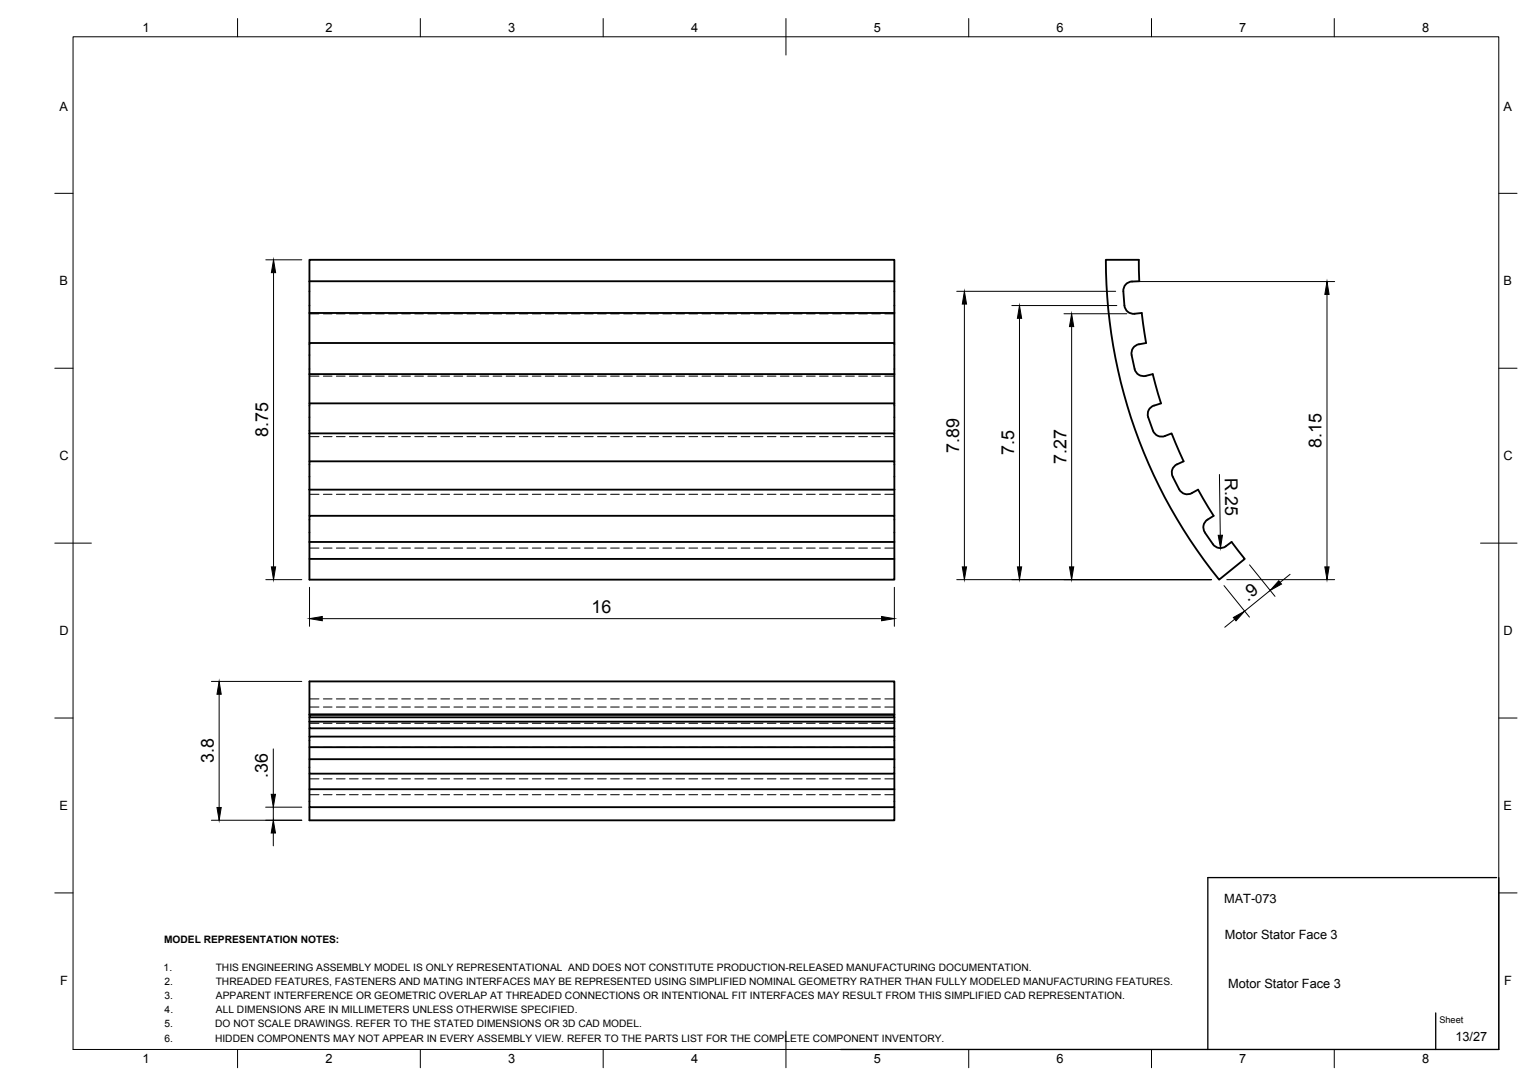
ISO-10303-21;
HEADER;
/* Generated by software containing ST-Developer
 * from STEP Tools, Inc. (www.steptools.com) 
 */

FILE_DESCRIPTION(
/* description */ ('CAx-IF Rec.Pracs.---Representation and Presentation of Product Manufa
cturing Information (PMI)---4.0---2014-10-13'),
/* implementation_level */ '2;1');

FILE_NAME(
/* name */ 'Motor Stator Face 3.step',
/* time_stamp */ '2026-10-24T18:52:33-07:00',
/* author */ (''),
/* organization */ (''),
/* preprocessor_version */ 'ST-DEVELOPER v20.2',
/* originating_system */ 'Autodesk Translation Framework v15.17.0.0',
/* authorisation */ '');

FILE_SCHEMA (('AP242_MANAGED_MODEL_BASED_3D_ENGINEERING_MIM_LF { 1 0 10303 442 2 1 4 }'));
ENDSEC;

DATA;
#10=MECHANICAL_DESIGN_GEOMETRIC_PRESENTATION_REPRESENTATION('',(#426),#34876);
#360=SHAPE_REPRESENTATION_RELATIONSHIP('SRR','None',#34997,#393);
#393=ADVANCED_BREP_SHAPE_REPRESENTATION('',(#459),#34855);
#426=STYLED_ITEM('',(#35163),#459);
#459=MANIFOLD_SOLID_BREP('Motor Stator Face 3',#19566);
#847=PLANE('',#21099);
#848=PLANE('',#21109);
#849=PLANE('',#21119);
#850=PLANE('',#21129);
#851=PLANE('',#21139);
#852=PLANE('',#21140);
#853=PLANE('',#21141);
#854=PLANE('',#21142);
#855=PLANE('',#21143);
#856=PLANE('',#21150);
#857=PLANE('',#21160);
#858=PLANE('',#21163);
#859=PLANE('',#21166);
#860=PLANE('',#21169);
#1841=LINE('',#31602,#3440);
#1842=LINE('',#31605,#3441);
#1843=LINE('',#31610,#3442);
#1844=LINE('',#31616,#3443);
#1845=LINE('',#31620,#3444);
#1846=LINE('',#31622,#3445);
#1847=LINE('',#31623,#3446);
#1848=LINE('',#31629,#3447);
#1849=LINE('',#31632,#3448);
#1850=LINE('',#31637,#3449);
#1851=LINE('',#31643,#3450);
#1852=LINE('',#31647,#3451);
#1853=LINE('',#31649,#3452);
#1854=LINE('',#31650,#3453);
#1855=LINE('',#31656,#3454);
#1856=LINE('',#31659,#3455);
#1857=LINE('',#31664,#3456);
#1858=LINE('',#31670,#3457);
#1859=LINE('',#31674,#3458);
#1860=LINE('',#31676,#3459);
#1861=LINE('',#31677,#3460);
#1862=LINE('',#31683,#3461);
#1863=LINE('',#31686,#3462);
#1864=LINE('',#31691,#3463);
#1865=LINE('',#31697,#3464);
#1866=LINE('',#31701,#3465);
#1867=LINE('',#31703,#3466);
#1868=LINE('',#31704,#3467);
#1869=LINE('',#31710,#3468);
#1870=LINE('',#31713,#3469);
#1871=LINE('',#31718,#3470);
#1872=LINE('',#31724,#3471);
#1873=LINE('',#31728,#3472);
#1874=LINE('',#31730,#3473);
#1875=LINE('',#31731,#3474);
#1876=LINE('',#31734,#3475);
#1877=LINE('',#31736,#3476);
#1878=LINE('',#31737,#3477);
#1879=LINE('',#31740,#3478);
#1880=LINE('',#31742,#3479);
#1881=LINE('',#31743,#3480);
#1882=LINE('',#31746,#3481);
#1883=LINE('',#31748,#3482);
#1884=LINE('',#31749,#3483);
#1885=LINE('',#31752,#3484);
#1886=LINE('',#31754,#3485);
#1887=LINE('',#31755,#3486);
#1888=LINE('',#31760,#3487);
#1889=LINE('',#31767,#3488);
#1890=LINE('',#31771,#3489);
#1891=LINE('',#31776,#3490);
#1892=LINE('',#31781,#3491);
#1893=LINE('',#31784,#3492);
#1894=LINE('',#31787,#3493);
#1895=LINE('',#31792,#3494);
#1896=LINE('',#31793,#3495);
#1897=LINE('',#31797,#3496);
#1898=LINE('',#31799,#3497);
#3440=VECTOR('',#25298,1.);
#3441=VECTOR('',#25301,1.);
#3442=VECTOR('',#25306,1.);
#3443=VECTOR('',#25313,1.);
#3444=VECTOR('',#25318,1.);
#3445=VECTOR('',#25319,1.);
#3446=VECTOR('',#25320,1.);
#3447=VECTOR('',#25325,1.);
#3448=VECTOR('',#25328,1.);
#3449=VECTOR('',#25333,1.);
#3450=VECTOR('',#25340,1.);
#3451=VECTOR('',#25345,1.);
#3452=VECTOR('',#25346,1.);
#3453=VECTOR('',#25347,1.);
#3454=VECTOR('',#25352,1.);
#3455=VECTOR('',#25355,1.);
#3456=VECTOR('',#25360,1.);
#3457=VECTOR('',#25367,1.);
#3458=VECTOR('',#25372,1.);
#3459=VECTOR('',#25373,1.);
#3460=VECTOR('',#25374,1.);
#3461=VECTOR('',#25379,1.);
#3462=VECTOR('',#25382,1.);
#3463=VECTOR('',#25387,1.);
#3464=VECTOR('',#25394,1.);
#3465=VECTOR('',#25399,1.);
#3466=VECTOR('',#25400,1.);
#3467=VECTOR('',#25401,1.);
#3468=VECTOR('',#25406,1.);
#3469=VECTOR('',#25409,1.);
#3470=VECTOR('',#25414,1.);
#3471=VECTOR('',#25421,1.);
#3472=VECTOR('',#25426,1.);
#3473=VECTOR('',#25427,1.);
#3474=VECTOR('',#25428,1.);
#3475=VECTOR('',#25431,1.);
#3476=VECTOR('',#25432,1.);
#3477=VECTOR('',#25433,1.);
#3478=VECTOR('',#25436,1.);
#3479=VECTOR('',#25437,1.);
#3480=VECTOR('',#25438,1.);
#3481=VECTOR('',#25441,1.);
#3482=VECTOR('',#25442,1.);
#3483=VECTOR('',#25443,1.);
#3484=VECTOR('',#25446,1.);
#3485=VECTOR('',#25447,1.);
#3486=VECTOR('',#25448,1.);
#3487=VECTOR('',#25453,1.);
#3488=VECTOR('',#25464,1.);
#3489=VECTOR('',#25467,1.);
#3490=VECTOR('',#25474,1.);
#3491=VECTOR('',#25481,1.);
#3492=VECTOR('',#25484,1.);
#3493=VECTOR('',#25489,1.);
#3494=VECTOR('',#25496,1.);
#3495=VECTOR('',#25497,1.);
#3496=VECTOR('',#25502,1.);
#3497=VECTOR('',#25505,1.);
#4525=CYLINDRICAL_SURFACE('',#21090,0.00025);
#4526=CYLINDRICAL_SURFACE('',#21093,0.01345);
#4527=CYLINDRICAL_SURFACE('',#21096,0.00025);
#4528=CYLINDRICAL_SURFACE('',#21100,0.00025);
#4529=CYLINDRICAL_SURFACE('',#21103,0.01345);
#4530=CYLINDRICAL_SURFACE('',#21106,0.00025);
#4531=CYLINDRICAL_SURFACE('',#21110,0.00025);
#4532=CYLINDRICAL_SURFACE('',#21113,0.01345);
#4533=CYLINDRICAL_SURFACE('',#21116,0.00025);
#4534=CYLINDRICAL_SURFACE('',#21120,0.00025);
#4535=CYLINDRICAL_SURFACE('',#21123,0.01345);
#4536=CYLINDRICAL_SURFACE('',#21126,0.00025);
#4537=CYLINDRICAL_SURFACE('',#21130,0.00025);
#4538=CYLINDRICAL_SURFACE('',#21133,0.01345);
#4539=CYLINDRICAL_SURFACE('',#21136,0.00025);
#4540=CYLINDRICAL_SURFACE('',#21144,0.013);
#4541=CYLINDRICAL_SURFACE('',#21147,0.013);
#4542=CYLINDRICAL_SURFACE('',#21156,0.013);
#4543=CYLINDRICAL_SURFACE('',#21158,0.013);
#4544=CYLINDRICAL_SURFACE('',#21161,0.013);
#4545=CYLINDRICAL_SURFACE('',#21164,0.0139);
#4546=CYLINDRICAL_SURFACE('',#21167,0.013);
#5309=FACE_OUTER_BOUND('',#6408,.T.);
#5310=FACE_OUTER_BOUND('',#6409,.T.);
#5311=FACE_OUTER_BOUND('',#6410,.T.);
#5312=FACE_OUTER_BOUND('',#6411,.T.);
#5313=FACE_OUTER_BOUND('',#6412,.T.);
#5314=FACE_OUTER_BOUND('',#6413,.T.);
#5315=FACE_OUTER_BOUND('',#6414,.T.);
#5316=FACE_OUTER_BOUND('',#6415,.T.);
#5317=FACE_OUTER_BOUND('',#6416,.T.);
#5318=FACE_OUTER_BOUND('',#6417,.T.);
#5319=FACE_OUTER_BOUND('',#6418,.T.);
#5320=FACE_OUTER_BOUND('',#6419,.T.);
#5321=FACE_OUTER_BOUND('',#6420,.T.);
#5322=FACE_OUTER_BOUND('',#6421,.T.);
#5323=FACE_OUTER_BOUND('',#6422,.T.);
#5324=FACE_OUTER_BOUND('',#6423,.T.);
#5325=FACE_OUTER_BOUND('',#6424,.T.);
#5326=FACE_OUTER_BOUND('',#6425,.T.);
#5327=FACE_OUTER_BOUND('',#6426,.T.);
#5328=FACE_OUTER_BOUND('',#6427,.T.);
#5329=FACE_OUTER_BOUND('',#6428,.T.);
#5330=FACE_OUTER_BOUND('',#6429,.T.);
#5331=FACE_OUTER_BOUND('',#6430,.T.);
#5332=FACE_OUTER_BOUND('',#6431,.T.);
#5333=FACE_OUTER_BOUND('',#6432,.T.);
#5334=FACE_OUTER_BOUND('',#6433,.T.);
#5335=FACE_OUTER_BOUND('',#6434,.T.);
#5336=FACE_OUTER_BOUND('',#6435,.T.);
#5337=FACE_OUTER_BOUND('',#6436,.T.);
#5338=FACE_OUTER_BOUND('',#6437,.T.);
#5339=FACE_OUTER_BOUND('',#6438,.T.);
#5340=FACE_OUTER_BOUND('',#6439,.T.);
#5341=FACE_OUTER_BOUND('',#6440,.T.);
#5342=FACE_OUTER_BOUND('',#6441,.T.);
#5343=FACE_OUTER_BOUND('',#6442,.T.);
#5344=FACE_OUTER_BOUND('',#6443,.T.);
#6408=EDGE_LOOP('',(#15580,#15581,#15582,#15583));
#6409=EDGE_LOOP('',(#15584,#15585,#15586,#15587));
#6410=EDGE_LOOP('',(#15588,#15589,#15590,#15591));
#6411=EDGE_LOOP('',(#15592,#15593,#15594,#15595));
#6412=EDGE_LOOP('',(#15596,#15597,#15598,#15599));
#6413=EDGE_LOOP('',(#15600,#15601,#15602,#15603));
#6414=EDGE_LOOP('',(#15604,#15605,#15606,#15607));
#6415=EDGE_LOOP('',(#15608,#15609,#15610,#15611));
#6416=EDGE_LOOP('',(#15612,#15613,#15614,#15615));
#6417=EDGE_LOOP('',(#15616,#15617,#15618,#15619));
#6418=EDGE_LOOP('',(#15620,#15621,#15622,#15623));
#6419=EDGE_LOOP('',(#15624,#15625,#15626,#15627));
#6420=EDGE_LOOP('',(#15628,#15629,#15630,#15631));
#6421=EDGE_LOOP('',(#15632,#15633,#15634,#15635));
#6422=EDGE_LOOP('',(#15636,#15637,#15638,#15639));
#6423=EDGE_LOOP('',(#15640,#15641,#15642,#15643));
#6424=EDGE_LOOP('',(#15644,#15645,#15646,#15647));
#6425=EDGE_LOOP('',(#15648,#15649,#15650,#15651));
#6426=EDGE_LOOP('',(#15652,#15653,#15654,#15655));
#6427=EDGE_LOOP('',(#15656,#15657,#15658,#15659));
#6428=EDGE_LOOP('',(#15660,#15661,#15662,#15663));
#6429=EDGE_LOOP('',(#15664,#15665,#15666,#15667));
#6430=EDGE_LOOP('',(#15668,#15669,#15670,#15671));
#6431=EDGE_LOOP('',(#15672,#15673,#15674,#15675));
#6432=EDGE_LOOP('',(#15676,#15677,#15678,#15679));
#6433=EDGE_LOOP('',(#15680,#15681,#15682,#15683));
#6434=EDGE_LOOP('',(#15684,#15685,#15686,#15687,#15688,#15689,#15690,#15691,
#15692,#15693,#15694,#15695,#15696,#15697,#15698,#15699,#15700,#15701,#15702,
#15703,#15704,#15705,#15706,#15707,#15708,#15709,#15710,#15711,#15712,#15713,
#15714,#15715,#15716,#15717));
#6435=EDGE_LOOP('',(#15718,#15719,#15720,#15721));
#6436=EDGE_LOOP('',(#15722,#15723,#15724,#15725));
#6437=EDGE_LOOP('',(#15726,#15727,#15728,#15729));
#6438=EDGE_LOOP('',(#15730,#15731,#15732,#15733));
#6439=EDGE_LOOP('',(#15734,#15735,#15736,#15737));
#6440=EDGE_LOOP('',(#15738,#15739,#15740,#15741));
#6441=EDGE_LOOP('',(#15742,#15743,#15744,#15745));
#6442=EDGE_LOOP('',(#15746,#15747,#15748,#15749));
#6443=EDGE_LOOP('',(#15750,#15751,#15752,#15753,#15754,#15755,#15756,#15757,
#15758,#15759,#15760,#15761,#15762,#15763,#15764,#15765,#15766,#15767,#15768,
#15769,#15770,#15771,#15772,#15773,#15774,#15775,#15776,#15777,#15778,#15779,
#15780,#15781,#15782,#15783));
#7490=CIRCLE('',#21091,0.000250000000013569);
#7491=CIRCLE('',#21092,0.000250000000013569);
#7492=CIRCLE('',#21094,0.0134500000000125);
#7493=CIRCLE('',#21095,0.0134500000000125);
#7494=CIRCLE('',#21097,0.000250000000013744);
#7495=CIRCLE('',#21098,0.000250000000013744);
#7496=CIRCLE('',#21101,0.000250000000013973);
#7497=CIRCLE('',#21102,0.000250000000013973);
#7498=CIRCLE('',#21104,0.0134500000000115);
#7499=CIRCLE('',#21105,0.0134500000000115);
#7500=CIRCLE('',#21107,0.000250000000014062);
#7501=CIRCLE('',#21108,0.000250000000014062);
#7502=CIRCLE('',#21111,0.000250000000014138);
#7503=CIRCLE('',#21112,0.000250000000014138);
#7504=CIRCLE('',#21114,0.0134500000000103);
#7505=CIRCLE('',#21115,0.0134500000000103);
#7506=CIRCLE('',#21117,0.000250000000014138);
#7507=CIRCLE('',#21118,0.000250000000014138);
#7508=CIRCLE('',#21121,0.000250000000014062);
#7509=CIRCLE('',#21122,0.000250000000014062);
#7510=CIRCLE('',#21124,0.0134500000000109);
#7511=CIRCLE('',#21125,0.0134500000000109);
#7512=CIRCLE('',#21127,0.000250000000013973);
#7513=CIRCLE('',#21128,0.000250000000013973);
#7514=CIRCLE('',#21131,0.000250000000013744);
#7515=CIRCLE('',#21132,0.000250000000013744);
#7516=CIRCLE('',#21134,0.013450000000012);
#7517=CIRCLE('',#21135,0.013450000000012);
#7518=CIRCLE('',#21137,0.000250000000013569);
#7519=CIRCLE('',#21138,0.000250000000013569);
#7520=CIRCLE('',#21145,0.0130000000000128);
#7521=CIRCLE('',#21146,0.0130000000000128);
#7522=CIRCLE('',#21148,0.0130000000000128);
#7523=CIRCLE('',#21149,0.0130000000000128);
#7524=CIRCLE('',#21151,0.0139000000000128);
#7525=CIRCLE('',#21152,0.0130000000000128);
#7526=CIRCLE('',#21153,0.0130000000000128);
#7527=CIRCLE('',#21154,0.0130000000000128);
#7528=CIRCLE('',#21155,0.0130000000000128);
#7529=CIRCLE('',#21157,0.0130000000000128);
#7530=CIRCLE('',#21159,0.0130000000000128);
#7531=CIRCLE('',#21162,0.0130000000000128);
#7532=CIRCLE('',#21165,0.0139000000000128);
#7533=CIRCLE('',#21168,0.0130000000000128);
#8990=VERTEX_POINT('',#31598);
#8991=VERTEX_POINT('',#31599);
#8992=VERTEX_POINT('',#31601);
#8993=VERTEX_POINT('',#31603);
#8994=VERTEX_POINT('',#31607);
#8995=VERTEX_POINT('',#31609);
#8996=VERTEX_POINT('',#31613);
#8997=VERTEX_POINT('',#31615);
#8998=VERTEX_POINT('',#31619);
#8999=VERTEX_POINT('',#31621);
#9000=VERTEX_POINT('',#31625);
#9001=VERTEX_POINT('',#31626);
#9002=VERTEX_POINT('',#31628);
#9003=VERTEX_POINT('',#31630);
#9004=VERTEX_POINT('',#31634);
#9005=VERTEX_POINT('',#31636);
#9006=VERTEX_POINT('',#31640);
#9007=VERTEX_POINT('',#31642);
#9008=VERTEX_POINT('',#31646);
#9009=VERTEX_POINT('',#31648);
#9010=VERTEX_POINT('',#31652);
#9011=VERTEX_POINT('',#31653);
#9012=VERTEX_POINT('',#31655);
#9013=VERTEX_POINT('',#31657);
#9014=VERTEX_POINT('',#31661);
#9015=VERTEX_POINT('',#31663);
#9016=VERTEX_POINT('',#31667);
#9017=VERTEX_POINT('',#31669);
#9018=VERTEX_POINT('',#31673);
#9019=VERTEX_POINT('',#31675);
#9020=VERTEX_POINT('',#31679);
#9021=VERTEX_POINT('',#31680);
#9022=VERTEX_POINT('',#31682);
#9023=VERTEX_POINT('',#31684);
#9024=VERTEX_POINT('',#31688);
#9025=VERTEX_POINT('',#31690);
#9026=VERTEX_POINT('',#31694);
#9027=VERTEX_POINT('',#31696);
#9028=VERTEX_POINT('',#31700);
#9029=VERTEX_POINT('',#31702);
#9030=VERTEX_POINT('',#31706);
#9031=VERTEX_POINT('',#31707);
#9032=VERTEX_POINT('',#31709);
#9033=VERTEX_POINT('',#31711);
#9034=VERTEX_POINT('',#31715);
#9035=VERTEX_POINT('',#31717);
#9036=VERTEX_POINT('',#31721);
#9037=VERTEX_POINT('',#31723);
#9038=VERTEX_POINT('',#31727);
#9039=VERTEX_POINT('',#31729);
#9040=VERTEX_POINT('',#31733);
#9041=VERTEX_POINT('',#31735);
#9042=VERTEX_POINT('',#31739);
#9043=VERTEX_POINT('',#31741);
#9044=VERTEX_POINT('',#31745);
#9045=VERTEX_POINT('',#31747);
#9046=VERTEX_POINT('',#31751);
#9047=VERTEX_POINT('',#31753);
#9048=VERTEX_POINT('',#31757);
#9049=VERTEX_POINT('',#31759);
#9050=VERTEX_POINT('',#31766);
#9051=VERTEX_POINT('',#31768);
#9052=VERTEX_POINT('',#31770);
#9053=VERTEX_POINT('',#31774);
#9054=VERTEX_POINT('',#31779);
#9055=VERTEX_POINT('',#31783);
#9056=VERTEX_POINT('',#31791);
#9057=VERTEX_POINT('',#31795);
#11348=EDGE_CURVE('',#8990,#8991,#7490,.T.);
#11349=EDGE_CURVE('',#8991,#8992,#1841,.T.);
#11350=EDGE_CURVE('',#8992,#8993,#7491,.T.);
#11351=EDGE_CURVE('',#8993,#8990,#1842,.T.);
#11352=EDGE_CURVE('',#8994,#8991,#7492,.T.);
#11353=EDGE_CURVE('',#8995,#8994,#1843,.T.);
#11354=EDGE_CURVE('',#8992,#8995,#7493,.T.);
#11355=EDGE_CURVE('',#8994,#8996,#7494,.T.);
#11356=EDGE_CURVE('',#8996,#8997,#1844,.T.);
#11357=EDGE_CURVE('',#8997,#8995,#7495,.T.);
#11358=EDGE_CURVE('',#8998,#8996,#1845,.T.);
#11359=EDGE_CURVE('',#8999,#8998,#1846,.T.);
#11360=EDGE_CURVE('',#8997,#8999,#1847,.T.);
#11361=EDGE_CURVE('',#9000,#9001,#7496,.T.);
#11362=EDGE_CURVE('',#9001,#9002,#1848,.T.);
#11363=EDGE_CURVE('',#9002,#9003,#7497,.T.);
#11364=EDGE_CURVE('',#9003,#9000,#1849,.T.);
#11365=EDGE_CURVE('',#9004,#9001,#7498,.T.);
#11366=EDGE_CURVE('',#9005,#9004,#1850,.T.);
#11367=EDGE_CURVE('',#9002,#9005,#7499,.T.);
#11368=EDGE_CURVE('',#9004,#9006,#7500,.T.);
#11369=EDGE_CURVE('',#9006,#9007,#1851,.T.);
#11370=EDGE_CURVE('',#9007,#9005,#7501,.T.);
#11371=EDGE_CURVE('',#9008,#9006,#1852,.T.);
#11372=EDGE_CURVE('',#9009,#9008,#1853,.T.);
#11373=EDGE_CURVE('',#9007,#9009,#1854,.T.);
#11374=EDGE_CURVE('',#9010,#9011,#7502,.T.);
#11375=EDGE_CURVE('',#9011,#9012,#1855,.T.);
#11376=EDGE_CURVE('',#9012,#9013,#7503,.T.);
#11377=EDGE_CURVE('',#9013,#9010,#1856,.T.);
#11378=EDGE_CURVE('',#9014,#9011,#7504,.T.);
#11379=EDGE_CURVE('',#9015,#9014,#1857,.T.);
#11380=EDGE_CURVE('',#9012,#9015,#7505,.T.);
#11381=EDGE_CURVE('',#9014,#9016,#7506,.T.);
#11382=EDGE_CURVE('',#9016,#9017,#1858,.T.);
#11383=EDGE_CURVE('',#9017,#9015,#7507,.T.);
#11384=EDGE_CURVE('',#9018,#9016,#1859,.T.);
#11385=EDGE_CURVE('',#9019,#9018,#1860,.T.);
#11386=EDGE_CURVE('',#9017,#9019,#1861,.T.);
#11387=EDGE_CURVE('',#9020,#9021,#7508,.T.);
#11388=EDGE_CURVE('',#9021,#9022,#1862,.T.);
#11389=EDGE_CURVE('',#9022,#9023,#7509,.T.);
#11390=EDGE_CURVE('',#9023,#9020,#1863,.T.);
#11391=EDGE_CURVE('',#9024,#9021,#7510,.T.);
#11392=EDGE_CURVE('',#9025,#9024,#1864,.T.);
#11393=EDGE_CURVE('',#9022,#9025,#7511,.T.);
#11394=EDGE_CURVE('',#9024,#9026,#7512,.T.);
#11395=EDGE_CURVE('',#9026,#9027,#1865,.T.);
#11396=EDGE_CURVE('',#9027,#9025,#7513,.T.);
#11397=EDGE_CURVE('',#9028,#9026,#1866,.T.);
#11398=EDGE_CURVE('',#9029,#9028,#1867,.T.);
#11399=EDGE_CURVE('',#9027,#9029,#1868,.T.);
#11400=EDGE_CURVE('',#9030,#9031,#7514,.T.);
#11401=EDGE_CURVE('',#9031,#9032,#1869,.T.);
#11402=EDGE_CURVE('',#9032,#9033,#7515,.T.);
#11403=EDGE_CURVE('',#9033,#9030,#1870,.T.);
#11404=EDGE_CURVE('',#9034,#9031,#7516,.T.);
#11405=EDGE_CURVE('',#9035,#9034,#1871,.T.);
#11406=EDGE_CURVE('',#9032,#9035,#7517,.T.);
#11407=EDGE_CURVE('',#9034,#9036,#7518,.T.);
#11408=EDGE_CURVE('',#9036,#9037,#1872,.T.);
#11409=EDGE_CURVE('',#9037,#9035,#7519,.T.);
#11410=EDGE_CURVE('',#9038,#9036,#1873,.T.);
#11411=EDGE_CURVE('',#9039,#9038,#1874,.T.);
#11412=EDGE_CURVE('',#9037,#9039,#1875,.T.);
#11413=EDGE_CURVE('',#9040,#9033,#1876,.T.);
#11414=EDGE_CURVE('',#9041,#9040,#1877,.T.);
#11415=EDGE_CURVE('',#9030,#9041,#1878,.T.);
#11416=EDGE_CURVE('',#9042,#9023,#1879,.T.);
#11417=EDGE_CURVE('',#9043,#9042,#1880,.T.);
#11418=EDGE_CURVE('',#9020,#9043,#1881,.T.);
#11419=EDGE_CURVE('',#9044,#9003,#1882,.T.);
#11420=EDGE_CURVE('',#9045,#9044,#1883,.T.);
#11421=EDGE_CURVE('',#9000,#9045,#1884,.T.);
#11422=EDGE_CURVE('',#9046,#8993,#1885,.T.);
#11423=EDGE_CURVE('',#9047,#9046,#1886,.T.);
#11424=EDGE_CURVE('',#8990,#9047,#1887,.T.);
#11425=EDGE_CURVE('',#9048,#9038,#7520,.T.);
#11426=EDGE_CURVE('',#9048,#9049,#1888,.T.);
#11427=EDGE_CURVE('',#9039,#9049,#7521,.T.);
#11428=EDGE_CURVE('',#9019,#9042,#7522,.T.);
#11429=EDGE_CURVE('',#9043,#9018,#7523,.T.);
#11430=EDGE_CURVE('',#9049,#9050,#1889,.T.);
#11431=EDGE_CURVE('',#9050,#9051,#7524,.T.);
#11432=EDGE_CURVE('',#9051,#9052,#1890,.T.);
#11433=EDGE_CURVE('',#9052,#9046,#7525,.T.);
#11434=EDGE_CURVE('',#8999,#9044,#7526,.T.);
#11435=EDGE_CURVE('',#9009,#9053,#7527,.T.);
#11436=EDGE_CURVE('',#9053,#9013,#1891,.T.);
#11437=EDGE_CURVE('',#9029,#9040,#7528,.T.);
#11438=EDGE_CURVE('',#9054,#9008,#7529,.T.);
#11439=EDGE_CURVE('',#9054,#9053,#1892,.T.);
#11440=EDGE_CURVE('',#9052,#9055,#1893,.T.);
#11441=EDGE_CURVE('',#9047,#9055,#7530,.T.);
#11442=EDGE_CURVE('',#9010,#9054,#1894,.T.);
#11443=EDGE_CURVE('',#9041,#9028,#7531,.T.);
#11444=EDGE_CURVE('',#9056,#9048,#1895,.T.);
#11445=EDGE_CURVE('',#9050,#9056,#1896,.T.);
#11446=EDGE_CURVE('',#9057,#9056,#7532,.T.);
#11447=EDGE_CURVE('',#9051,#9057,#1897,.T.);
#11448=EDGE_CURVE('',#9055,#9057,#1898,.T.);
#11449=EDGE_CURVE('',#9045,#8998,#7533,.T.);
#15580=ORIENTED_EDGE('',*,*,#11348,.T.);
#15581=ORIENTED_EDGE('',*,*,#11349,.T.);
#15582=ORIENTED_EDGE('',*,*,#11350,.T.);
#15583=ORIENTED_EDGE('',*,*,#11351,.T.);
#15584=ORIENTED_EDGE('',*,*,#11349,.F.);
#15585=ORIENTED_EDGE('',*,*,#11352,.F.);
#15586=ORIENTED_EDGE('',*,*,#11353,.F.);
#15587=ORIENTED_EDGE('',*,*,#11354,.F.);
#15588=ORIENTED_EDGE('',*,*,#11355,.T.);
#15589=ORIENTED_EDGE('',*,*,#11356,.T.);
#15590=ORIENTED_EDGE('',*,*,#11357,.T.);
#15591=ORIENTED_EDGE('',*,*,#11353,.T.);
#15592=ORIENTED_EDGE('',*,*,#11356,.F.);
#15593=ORIENTED_EDGE('',*,*,#11358,.F.);
#15594=ORIENTED_EDGE('',*,*,#11359,.F.);
#15595=ORIENTED_EDGE('',*,*,#11360,.F.);
#15596=ORIENTED_EDGE('',*,*,#11361,.T.);
#15597=ORIENTED_EDGE('',*,*,#11362,.T.);
#15598=ORIENTED_EDGE('',*,*,#11363,.T.);
#15599=ORIENTED_EDGE('',*,*,#11364,.T.);
#15600=ORIENTED_EDGE('',*,*,#11362,.F.);
#15601=ORIENTED_EDGE('',*,*,#11365,.F.);
#15602=ORIENTED_EDGE('',*,*,#11366,.F.);
#15603=ORIENTED_EDGE('',*,*,#11367,.F.);
#15604=ORIENTED_EDGE('',*,*,#11368,.T.);
#15605=ORIENTED_EDGE('',*,*,#11369,.T.);
#15606=ORIENTED_EDGE('',*,*,#11370,.T.);
#15607=ORIENTED_EDGE('',*,*,#11366,.T.);
#15608=ORIENTED_EDGE('',*,*,#11369,.F.);
#15609=ORIENTED_EDGE('',*,*,#11371,.F.);
#15610=ORIENTED_EDGE('',*,*,#11372,.F.);
#15611=ORIENTED_EDGE('',*,*,#11373,.F.);
#15612=ORIENTED_EDGE('',*,*,#11374,.T.);
#15613=ORIENTED_EDGE('',*,*,#11375,.T.);
#15614=ORIENTED_EDGE('',*,*,#11376,.T.);
#15615=ORIENTED_EDGE('',*,*,#11377,.T.);
#15616=ORIENTED_EDGE('',*,*,#11375,.F.);
#15617=ORIENTED_EDGE('',*,*,#11378,.F.);
#15618=ORIENTED_EDGE('',*,*,#11379,.F.);
#15619=ORIENTED_EDGE('',*,*,#11380,.F.);
#15620=ORIENTED_EDGE('',*,*,#11381,.T.);
#15621=ORIENTED_EDGE('',*,*,#11382,.T.);
#15622=ORIENTED_EDGE('',*,*,#11383,.T.);
#15623=ORIENTED_EDGE('',*,*,#11379,.T.);
#15624=ORIENTED_EDGE('',*,*,#11382,.F.);
#15625=ORIENTED_EDGE('',*,*,#11384,.F.);
#15626=ORIENTED_EDGE('',*,*,#11385,.F.);
#15627=ORIENTED_EDGE('',*,*,#11386,.F.);
#15628=ORIENTED_EDGE('',*,*,#11387,.T.);
#15629=ORIENTED_EDGE('',*,*,#11388,.T.);
#15630=ORIENTED_EDGE('',*,*,#11389,.T.);
#15631=ORIENTED_EDGE('',*,*,#11390,.T.);
#15632=ORIENTED_EDGE('',*,*,#11388,.F.);
#15633=ORIENTED_EDGE('',*,*,#11391,.F.);
#15634=ORIENTED_EDGE('',*,*,#11392,.F.);
#15635=ORIENTED_EDGE('',*,*,#11393,.F.);
#15636=ORIENTED_EDGE('',*,*,#11394,.T.);
#15637=ORIENTED_EDGE('',*,*,#11395,.T.);
#15638=ORIENTED_EDGE('',*,*,#11396,.T.);
#15639=ORIENTED_EDGE('',*,*,#11392,.T.);
#15640=ORIENTED_EDGE('',*,*,#11395,.F.);
#15641=ORIENTED_EDGE('',*,*,#11397,.F.);
#15642=ORIENTED_EDGE('',*,*,#11398,.F.);
#15643=ORIENTED_EDGE('',*,*,#11399,.F.);
#15644=ORIENTED_EDGE('',*,*,#11400,.T.);
#15645=ORIENTED_EDGE('',*,*,#11401,.T.);
#15646=ORIENTED_EDGE('',*,*,#11402,.T.);
#15647=ORIENTED_EDGE('',*,*,#11403,.T.);
#15648=ORIENTED_EDGE('',*,*,#11401,.F.);
#15649=ORIENTED_EDGE('',*,*,#11404,.F.);
#15650=ORIENTED_EDGE('',*,*,#11405,.F.);
#15651=ORIENTED_EDGE('',*,*,#11406,.F.);
#15652=ORIENTED_EDGE('',*,*,#11407,.T.);
#15653=ORIENTED_EDGE('',*,*,#11408,.T.);
#15654=ORIENTED_EDGE('',*,*,#11409,.T.);
#15655=ORIENTED_EDGE('',*,*,#11405,.T.);
#15656=ORIENTED_EDGE('',*,*,#11408,.F.);
#15657=ORIENTED_EDGE('',*,*,#11410,.F.);
#15658=ORIENTED_EDGE('',*,*,#11411,.F.);
#15659=ORIENTED_EDGE('',*,*,#11412,.F.);
#15660=ORIENTED_EDGE('',*,*,#11403,.F.);
#15661=ORIENTED_EDGE('',*,*,#11413,.F.);
#15662=ORIENTED_EDGE('',*,*,#11414,.F.);
#15663=ORIENTED_EDGE('',*,*,#11415,.F.);
#15664=ORIENTED_EDGE('',*,*,#11390,.F.);
#15665=ORIENTED_EDGE('',*,*,#11416,.F.);
#15666=ORIENTED_EDGE('',*,*,#11417,.F.);
#15667=ORIENTED_EDGE('',*,*,#11418,.F.);
#15668=ORIENTED_EDGE('',*,*,#11364,.F.);
#15669=ORIENTED_EDGE('',*,*,#11419,.F.);
#15670=ORIENTED_EDGE('',*,*,#11420,.F.);
#15671=ORIENTED_EDGE('',*,*,#11421,.F.);
#15672=ORIENTED_EDGE('',*,*,#11351,.F.);
#15673=ORIENTED_EDGE('',*,*,#11422,.F.);
#15674=ORIENTED_EDGE('',*,*,#11423,.F.);
#15675=ORIENTED_EDGE('',*,*,#11424,.F.);
#15676=ORIENTED_EDGE('',*,*,#11411,.T.);
#15677=ORIENTED_EDGE('',*,*,#11425,.F.);
#15678=ORIENTED_EDGE('',*,*,#11426,.T.);
#15679=ORIENTED_EDGE('',*,*,#11427,.F.);
#15680=ORIENTED_EDGE('',*,*,#11417,.T.);
#15681=ORIENTED_EDGE('',*,*,#11428,.F.);
#15682=ORIENTED_EDGE('',*,*,#11385,.T.);
#15683=ORIENTED_EDGE('',*,*,#11429,.F.);
#15684=ORIENTED_EDGE('',*,*,#11413,.T.);
#15685=ORIENTED_EDGE('',*,*,#11402,.F.);
#15686=ORIENTED_EDGE('',*,*,#11406,.T.);
#15687=ORIENTED_EDGE('',*,*,#11409,.F.);
#15688=ORIENTED_EDGE('',*,*,#11412,.T.);
#15689=ORIENTED_EDGE('',*,*,#11427,.T.);
#15690=ORIENTED_EDGE('',*,*,#11430,.T.);
#15691=ORIENTED_EDGE('',*,*,#11431,.T.);
#15692=ORIENTED_EDGE('',*,*,#11432,.T.);
#15693=ORIENTED_EDGE('',*,*,#11433,.T.);
#15694=ORIENTED_EDGE('',*,*,#11422,.T.);
#15695=ORIENTED_EDGE('',*,*,#11350,.F.);
#15696=ORIENTED_EDGE('',*,*,#11354,.T.);
#15697=ORIENTED_EDGE('',*,*,#11357,.F.);
#15698=ORIENTED_EDGE('',*,*,#11360,.T.);
#15699=ORIENTED_EDGE('',*,*,#11434,.T.);
#15700=ORIENTED_EDGE('',*,*,#11419,.T.);
#15701=ORIENTED_EDGE('',*,*,#11363,.F.);
#15702=ORIENTED_EDGE('',*,*,#11367,.T.);
#15703=ORIENTED_EDGE('',*,*,#11370,.F.);
#15704=ORIENTED_EDGE('',*,*,#11373,.T.);
#15705=ORIENTED_EDGE('',*,*,#11435,.T.);
#15706=ORIENTED_EDGE('',*,*,#11436,.T.);
#15707=ORIENTED_EDGE('',*,*,#11376,.F.);
#15708=ORIENTED_EDGE('',*,*,#11380,.T.);
#15709=ORIENTED_EDGE('',*,*,#11383,.F.);
#15710=ORIENTED_EDGE('',*,*,#11386,.T.);
#15711=ORIENTED_EDGE('',*,*,#11428,.T.);
#15712=ORIENTED_EDGE('',*,*,#11416,.T.);
#15713=ORIENTED_EDGE('',*,*,#11389,.F.);
#15714=ORIENTED_EDGE('',*,*,#11393,.T.);
#15715=ORIENTED_EDGE('',*,*,#11396,.F.);
#15716=ORIENTED_EDGE('',*,*,#11399,.T.);
#15717=ORIENTED_EDGE('',*,*,#11437,.T.);
#15718=ORIENTED_EDGE('',*,*,#11372,.T.);
#15719=ORIENTED_EDGE('',*,*,#11438,.F.);
#15720=ORIENTED_EDGE('',*,*,#11439,.T.);
#15721=ORIENTED_EDGE('',*,*,#11435,.F.);
#15722=ORIENTED_EDGE('',*,*,#11423,.T.);
#15723=ORIENTED_EDGE('',*,*,#11433,.F.);
#15724=ORIENTED_EDGE('',*,*,#11440,.T.);
#15725=ORIENTED_EDGE('',*,*,#11441,.F.);
#15726=ORIENTED_EDGE('',*,*,#11377,.F.);
#15727=ORIENTED_EDGE('',*,*,#11436,.F.);
#15728=ORIENTED_EDGE('',*,*,#11439,.F.);
#15729=ORIENTED_EDGE('',*,*,#11442,.F.);
#15730=ORIENTED_EDGE('',*,*,#11414,.T.);
#15731=ORIENTED_EDGE('',*,*,#11437,.F.);
#15732=ORIENTED_EDGE('',*,*,#11398,.T.);
#15733=ORIENTED_EDGE('',*,*,#11443,.F.);
#15734=ORIENTED_EDGE('',*,*,#11426,.F.);
#15735=ORIENTED_EDGE('',*,*,#11444,.F.);
#15736=ORIENTED_EDGE('',*,*,#11445,.F.);
#15737=ORIENTED_EDGE('',*,*,#11430,.F.);
#15738=ORIENTED_EDGE('',*,*,#11445,.T.);
#15739=ORIENTED_EDGE('',*,*,#11446,.F.);
#15740=ORIENTED_EDGE('',*,*,#11447,.F.);
#15741=ORIENTED_EDGE('',*,*,#11431,.F.);
#15742=ORIENTED_EDGE('',*,*,#11447,.T.);
#15743=ORIENTED_EDGE('',*,*,#11448,.F.);
#15744=ORIENTED_EDGE('',*,*,#11440,.F.);
#15745=ORIENTED_EDGE('',*,*,#11432,.F.);
#15746=ORIENTED_EDGE('',*,*,#11420,.T.);
#15747=ORIENTED_EDGE('',*,*,#11434,.F.);
#15748=ORIENTED_EDGE('',*,*,#11359,.T.);
#15749=ORIENTED_EDGE('',*,*,#11449,.F.);
#15750=ORIENTED_EDGE('',*,*,#11415,.T.);
#15751=ORIENTED_EDGE('',*,*,#11443,.T.);
#15752=ORIENTED_EDGE('',*,*,#11397,.T.);
#15753=ORIENTED_EDGE('',*,*,#11394,.F.);
#15754=ORIENTED_EDGE('',*,*,#11391,.T.);
#15755=ORIENTED_EDGE('',*,*,#11387,.F.);
#15756=ORIENTED_EDGE('',*,*,#11418,.T.);
#15757=ORIENTED_EDGE('',*,*,#11429,.T.);
#15758=ORIENTED_EDGE('',*,*,#11384,.T.);
#15759=ORIENTED_EDGE('',*,*,#11381,.F.);
#15760=ORIENTED_EDGE('',*,*,#11378,.T.);
#15761=ORIENTED_EDGE('',*,*,#11374,.F.);
#15762=ORIENTED_EDGE('',*,*,#11442,.T.);
#15763=ORIENTED_EDGE('',*,*,#11438,.T.);
#15764=ORIENTED_EDGE('',*,*,#11371,.T.);
#15765=ORIENTED_EDGE('',*,*,#11368,.F.);
#15766=ORIENTED_EDGE('',*,*,#11365,.T.);
#15767=ORIENTED_EDGE('',*,*,#11361,.F.);
#15768=ORIENTED_EDGE('',*,*,#11421,.T.);
#15769=ORIENTED_EDGE('',*,*,#11449,.T.);
#15770=ORIENTED_EDGE('',*,*,#11358,.T.);
#15771=ORIENTED_EDGE('',*,*,#11355,.F.);
#15772=ORIENTED_EDGE('',*,*,#11352,.T.);
#15773=ORIENTED_EDGE('',*,*,#11348,.F.);
#15774=ORIENTED_EDGE('',*,*,#11424,.T.);
#15775=ORIENTED_EDGE('',*,*,#11441,.T.);
#15776=ORIENTED_EDGE('',*,*,#11448,.T.);
#15777=ORIENTED_EDGE('',*,*,#11446,.T.);
#15778=ORIENTED_EDGE('',*,*,#11444,.T.);
#15779=ORIENTED_EDGE('',*,*,#11425,.T.);
#15780=ORIENTED_EDGE('',*,*,#11410,.T.);
#15781=ORIENTED_EDGE('',*,*,#11407,.F.);
#15782=ORIENTED_EDGE('',*,*,#11404,.T.);
#15783=ORIENTED_EDGE('',*,*,#11400,.F.);
#19025=ADVANCED_FACE('',(#5309),#4525,.F.);
#19026=ADVANCED_FACE('',(#5310),#4526,.F.);
#19027=ADVANCED_FACE('',(#5311),#4527,.F.);
#19028=ADVANCED_FACE('',(#5312),#847,.F.);
#19029=ADVANCED_FACE('',(#5313),#4528,.F.);
#19030=ADVANCED_FACE('',(#5314),#4529,.F.);
#19031=ADVANCED_FACE('',(#5315),#4530,.F.);
#19032=ADVANCED_FACE('',(#5316),#848,.F.);
#19033=ADVANCED_FACE('',(#5317),#4531,.F.);
#19034=ADVANCED_FACE('',(#5318),#4532,.F.);
#19035=ADVANCED_FACE('',(#5319),#4533,.F.);
#19036=ADVANCED_FACE('',(#5320),#849,.F.);
#19037=ADVANCED_FACE('',(#5321),#4534,.F.);
#19038=ADVANCED_FACE('',(#5322),#4535,.F.);
#19039=ADVANCED_FACE('',(#5323),#4536,.F.);
#19040=ADVANCED_FACE('',(#5324),#850,.F.);
#19041=ADVANCED_FACE('',(#5325),#4537,.F.);
#19042=ADVANCED_FACE('',(#5326),#4538,.F.);
#19043=ADVANCED_FACE('',(#5327),#4539,.F.);
#19044=ADVANCED_FACE('',(#5328),#851,.F.);
#19045=ADVANCED_FACE('',(#5329),#852,.F.);
#19046=ADVANCED_FACE('',(#5330),#853,.F.);
#19047=ADVANCED_FACE('',(#5331),#854,.F.);
#19048=ADVANCED_FACE('',(#5332),#855,.F.);
#19049=ADVANCED_FACE('',(#5333),#4540,.F.);
#19050=ADVANCED_FACE('',(#5334),#4541,.F.);
#19051=ADVANCED_FACE('',(#5335),#856,.F.);
#19052=ADVANCED_FACE('',(#5336),#4542,.F.);
#19053=ADVANCED_FACE('',(#5337),#4543,.F.);
#19054=ADVANCED_FACE('',(#5338),#857,.F.);
#19055=ADVANCED_FACE('',(#5339),#4544,.F.);
#19056=ADVANCED_FACE('',(#5340),#858,.T.);
#19057=ADVANCED_FACE('',(#5341),#4545,.T.);
#19058=ADVANCED_FACE('',(#5342),#859,.T.);
#19059=ADVANCED_FACE('',(#5343),#4546,.F.);
#19060=ADVANCED_FACE('',(#5344),#860,.T.);
#19566=CLOSED_SHELL('',(#19025,#19026,#19027,#19028,#19029,#19030,#19031,
#19032,#19033,#19034,#19035,#19036,#19037,#19038,#19039,#19040,#19041,#19042,
#19043,#19044,#19045,#19046,#19047,#19048,#19049,#19050,#19051,#19052,#19053,
#19054,#19055,#19056,#19057,#19058,#19059,#19060));
#21089=AXIS2_PLACEMENT_3D('',#31596,#25292,#25293);
#21090=AXIS2_PLACEMENT_3D('',#31597,#25294,#25295);
#21091=AXIS2_PLACEMENT_3D('',#31600,#25296,#25297);
#21092=AXIS2_PLACEMENT_3D('',#31604,#25299,#25300);
#21093=AXIS2_PLACEMENT_3D('',#31606,#25302,#25303);
#21094=AXIS2_PLACEMENT_3D('',#31608,#25304,#25305);
#21095=AXIS2_PLACEMENT_3D('',#31611,#25307,#25308);
#21096=AXIS2_PLACEMENT_3D('',#31612,#25309,#25310);
#21097=AXIS2_PLACEMENT_3D('',#31614,#25311,#25312);
#21098=AXIS2_PLACEMENT_3D('',#31617,#25314,#25315);
#21099=AXIS2_PLACEMENT_3D('',#31618,#25316,#25317);
#21100=AXIS2_PLACEMENT_3D('',#31624,#25321,#25322);
#21101=AXIS2_PLACEMENT_3D('',#31627,#25323,#25324);
#21102=AXIS2_PLACEMENT_3D('',#31631,#25326,#25327);
#21103=AXIS2_PLACEMENT_3D('',#31633,#25329,#25330);
#21104=AXIS2_PLACEMENT_3D('',#31635,#25331,#25332);
#21105=AXIS2_PLACEMENT_3D('',#31638,#25334,#25335);
#21106=AXIS2_PLACEMENT_3D('',#31639,#25336,#25337);
#21107=AXIS2_PLACEMENT_3D('',#31641,#25338,#25339);
#21108=AXIS2_PLACEMENT_3D('',#31644,#25341,#25342);
#21109=AXIS2_PLACEMENT_3D('',#31645,#25343,#25344);
#21110=AXIS2_PLACEMENT_3D('',#31651,#25348,#25349);
#21111=AXIS2_PLACEMENT_3D('',#31654,#25350,#25351);
#21112=AXIS2_PLACEMENT_3D('',#31658,#25353,#25354);
#21113=AXIS2_PLACEMENT_3D('',#31660,#25356,#25357);
#21114=AXIS2_PLACEMENT_3D('',#31662,#25358,#25359);
#21115=AXIS2_PLACEMENT_3D('',#31665,#25361,#25362);
#21116=AXIS2_PLACEMENT_3D('',#31666,#25363,#25364);
#21117=AXIS2_PLACEMENT_3D('',#31668,#25365,#25366);
#21118=AXIS2_PLACEMENT_3D('',#31671,#25368,#25369);
#21119=AXIS2_PLACEMENT_3D('',#31672,#25370,#25371);
#21120=AXIS2_PLACEMENT_3D('',#31678,#25375,#25376);
#21121=AXIS2_PLACEMENT_3D('',#31681,#25377,#25378);
#21122=AXIS2_PLACEMENT_3D('',#31685,#25380,#25381);
#21123=AXIS2_PLACEMENT_3D('',#31687,#25383,#25384);
#21124=AXIS2_PLACEMENT_3D('',#31689,#25385,#25386);
#21125=AXIS2_PLACEMENT_3D('',#31692,#25388,#25389);
#21126=AXIS2_PLACEMENT_3D('',#31693,#25390,#25391);
#21127=AXIS2_PLACEMENT_3D('',#31695,#25392,#25393);
#21128=AXIS2_PLACEMENT_3D('',#31698,#25395,#25396);
#21129=AXIS2_PLACEMENT_3D('',#31699,#25397,#25398);
#21130=AXIS2_PLACEMENT_3D('',#31705,#25402,#25403);
#21131=AXIS2_PLACEMENT_3D('',#31708,#25404,#25405);
#21132=AXIS2_PLACEMENT_3D('',#31712,#25407,#25408);
#21133=AXIS2_PLACEMENT_3D('',#31714,#25410,#25411);
#21134=AXIS2_PLACEMENT_3D('',#31716,#25412,#25413);
#21135=AXIS2_PLACEMENT_3D('',#31719,#25415,#25416);
#21136=AXIS2_PLACEMENT_3D('',#31720,#25417,#25418);
#21137=AXIS2_PLACEMENT_3D('',#31722,#25419,#25420);
#21138=AXIS2_PLACEMENT_3D('',#31725,#25422,#25423);
#21139=AXIS2_PLACEMENT_3D('',#31726,#25424,#25425);
#21140=AXIS2_PLACEMENT_3D('',#31732,#25429,#25430);
#21141=AXIS2_PLACEMENT_3D('',#31738,#25434,#25435);
#21142=AXIS2_PLACEMENT_3D('',#31744,#25439,#25440);
#21143=AXIS2_PLACEMENT_3D('',#31750,#25444,#25445);
#21144=AXIS2_PLACEMENT_3D('',#31756,#25449,#25450);
#21145=AXIS2_PLACEMENT_3D('',#31758,#25451,#25452);
#21146=AXIS2_PLACEMENT_3D('',#31761,#25454,#25455);
#21147=AXIS2_PLACEMENT_3D('',#31762,#25456,#25457);
#21148=AXIS2_PLACEMENT_3D('',#31763,#25458,#25459);
#21149=AXIS2_PLACEMENT_3D('',#31764,#25460,#25461);
#21150=AXIS2_PLACEMENT_3D('',#31765,#25462,#25463);
#21151=AXIS2_PLACEMENT_3D('',#31769,#25465,#25466);
#21152=AXIS2_PLACEMENT_3D('',#31772,#25468,#25469);
#21153=AXIS2_PLACEMENT_3D('',#31773,#25470,#25471);
#21154=AXIS2_PLACEMENT_3D('',#31775,#25472,#25473);
#21155=AXIS2_PLACEMENT_3D('',#31777,#25475,#25476);
#21156=AXIS2_PLACEMENT_3D('',#31778,#25477,#25478);
#21157=AXIS2_PLACEMENT_3D('',#31780,#25479,#25480);
#21158=AXIS2_PLACEMENT_3D('',#31782,#25482,#25483);
#21159=AXIS2_PLACEMENT_3D('',#31785,#25485,#25486);
#21160=AXIS2_PLACEMENT_3D('',#31786,#25487,#25488);
#21161=AXIS2_PLACEMENT_3D('',#31788,#25490,#25491);
#21162=AXIS2_PLACEMENT_3D('',#31789,#25492,#25493);
#21163=AXIS2_PLACEMENT_3D('',#31790,#25494,#25495);
#21164=AXIS2_PLACEMENT_3D('',#31794,#25498,#25499);
#21165=AXIS2_PLACEMENT_3D('',#31796,#25500,#25501);
#21166=AXIS2_PLACEMENT_3D('',#31798,#25503,#25504);
#21167=AXIS2_PLACEMENT_3D('',#31800,#25506,#25507);
#21168=AXIS2_PLACEMENT_3D('',#31801,#25508,#25509);
#21169=AXIS2_PLACEMENT_3D('',#31802,#25510,#25511);
#25292=DIRECTION('axis',(0.,0.,1.));
#25293=DIRECTION('refdir',(1.,0.,0.));
#25294=DIRECTION('center_axis',(0.,-1.,0.));
#25295=DIRECTION('ref_axis',(-0.479079334165917,0.,-0.877771605587206));
#25296=DIRECTION('center_axis',(0.,1.,0.));
#25297=DIRECTION('ref_axis',(-0.479079334179915,0.,-0.877771605579566));
#25298=DIRECTION('',(0.,-1.,0.));
#25299=DIRECTION('center_axis',(0.,-1.,0.));
#25300=DIRECTION('ref_axis',(-0.479079334179915,0.,-0.877771605579566));
#25301=DIRECTION('',(0.,1.,0.));
#25302=DIRECTION('center_axis',(0.,-1.,0.));
#25303=DIRECTION('ref_axis',(-0.956725679001189,0.,-0.290991366091358));
#25304=DIRECTION('center_axis',(0.,-1.,0.));
#25305=DIRECTION('ref_axis',(-0.956725679001045,0.,-0.290991366091831));
#25306=DIRECTION('',(0.,1.,0.));
#25307=DIRECTION('center_axis',(0.,1.,0.));
#25308=DIRECTION('ref_axis',(-0.956725679001045,0.,-0.290991366091831));
#25309=DIRECTION('center_axis',(0.,-1.,0.));
#25310=DIRECTION('ref_axis',(-0.853780676609416,0.,0.520632842076226));
#25311=DIRECTION('center_axis',(0.,1.,0.));
#25312=DIRECTION('ref_axis',(-0.853780676602478,0.,0.520632842087603));
#25313=DIRECTION('',(0.,-1.,0.));
#25314=DIRECTION('center_axis',(0.,-1.,0.));
#25315=DIRECTION('ref_axis',(-0.853780676602478,0.,0.520632842087603));
#25316=DIRECTION('center_axis',(-0.22635692418354,0.,0.974044425513625));
#25317=DIRECTION('ref_axis',(0.,1.,0.));
#25318=DIRECTION('',(-0.974044425513455,0.,-0.226356924184268));
#25319=DIRECTION('',(0.,1.,0.));
#25320=DIRECTION('',(0.974044425513455,0.,0.226356924184268));
#25321=DIRECTION('center_axis',(0.,-1.,0.));
#25322=DIRECTION('ref_axis',(-0.589552929365357,0.,-0.807729746559285));
#25323=DIRECTION('center_axis',(0.,1.,0.));
#25324=DIRECTION('ref_axis',(-0.589552929372406,0.,-0.80772974655414));
#25325=DIRECTION('',(0.,-1.,0.));
#25326=DIRECTION('center_axis',(0.,-1.,0.));
#25327=DIRECTION('ref_axis',(-0.589552929372406,0.,-0.80772974655414));
#25328=DIRECTION('',(0.,1.,0.));
#25329=DIRECTION('center_axis',(0.,-1.,0.));
#25330=DIRECTION('ref_axis',(-0.986522753174914,0.,-0.163624134736254));
#25331=DIRECTION('center_axis',(0.,-1.,0.));
#25332=DIRECTION('ref_axis',(-0.986522753174814,0.,-0.163624134736857));
#25333=DIRECTION('',(0.,1.,0.));
#25334=DIRECTION('center_axis',(0.,1.,0.));
#25335=DIRECTION('ref_axis',(-0.986522753174814,0.,-0.163624134736857));
#25336=DIRECTION('center_axis',(0.,-1.,0.));
#25337=DIRECTION('ref_axis',(-0.778520242143747,0.,0.627619496647803));
#25338=DIRECTION('center_axis',(0.,1.,0.));
#25339=DIRECTION('ref_axis',(-0.778520242139959,0.,0.627619496652502));
#25340=DIRECTION('',(0.,-1.,0.));
#25341=DIRECTION('center_axis',(0.,-1.,0.));
#25342=DIRECTION('ref_axis',(-0.778520242139959,0.,0.627619496652502));
#25343=DIRECTION('center_axis',(-0.0972820994026906,0.,0.995256847821609));
#25344=DIRECTION('ref_axis',(0.,1.,0.));
#25345=DIRECTION('',(-0.995256847821522,0.,-0.0972820994035843));
#25346=DIRECTION('',(0.,1.,0.));
#25347=DIRECTION('',(0.995256847821522,0.,0.0972820994035843));
#25348=DIRECTION('center_axis',(0.,-1.,0.));
#25349=DIRECTION('ref_axis',(-0.689939110488408,0.,-0.723867407622739));
#25350=DIRECTION('center_axis',(0.,1.,0.));
#25351=DIRECTION('ref_axis',(-0.689939110489391,0.,-0.723867407621802));
#25352=DIRECTION('',(0.,-1.,0.));
#25353=DIRECTION('center_axis',(0.,-1.,0.));
#25354=DIRECTION('ref_axis',(-0.689939110489391,0.,-0.723867407621802));
#25355=DIRECTION('',(0.,1.,0.));
#25356=DIRECTION('center_axis',(0.,-1.,0.));
#25357=DIRECTION('ref_axis',(-0.999440149526036,0.,-0.0334572490706319));
#25358=DIRECTION('center_axis',(0.,-1.,0.));
#25359=DIRECTION('ref_axis',(-0.999440149526012,0.,-0.0334572490713497));
#25360=DIRECTION('',(0.,1.,0.));
#25361=DIRECTION('center_axis',(0.,1.,0.));
#25362=DIRECTION('ref_axis',(-0.999440149526012,0.,-0.0334572490713497));
#25363=DIRECTION('center_axis',(0.,-1.,0.));
#25364=DIRECTION('ref_axis',(-0.689939110488409,0.,0.723867407622738));
#25365=DIRECTION('center_axis',(0.,1.,0.));
#25366=DIRECTION('ref_axis',(-0.689939110489391,0.,0.723867407621802));
#25367=DIRECTION('',(0.,-1.,0.));
#25368=DIRECTION('center_axis',(0.,-1.,0.));
#25369=DIRECTION('ref_axis',(-0.689939110489391,0.,0.723867407621802));
#25370=DIRECTION('center_axis',(0.0334572490706321,0.,0.999440149526036));
#25371=DIRECTION('ref_axis',(0.,-1.,0.));
#25372=DIRECTION('',(-0.999440149526004,0.,0.0334572490715975));
#25373=DIRECTION('',(0.,1.,0.));
#25374=DIRECTION('',(0.999440149526004,0.,-0.0334572490715975));
#25375=DIRECTION('center_axis',(0.,-1.,0.));
#25376=DIRECTION('ref_axis',(-0.778520242143747,0.,-0.627619496647803));
#25377=DIRECTION('center_axis',(0.,1.,0.));
#25378=DIRECTION('ref_axis',(-0.778520242139959,0.,-0.627619496652502));
#25379=DIRECTION('',(0.,-1.,0.));
#25380=DIRECTION('center_axis',(0.,-1.,0.));
#25381=DIRECTION('ref_axis',(-0.778520242139959,0.,-0.627619496652502));
#25382=DIRECTION('',(0.,1.,0.));
#25383=DIRECTION('center_axis',(0.,-1.,0.));
#25384=DIRECTION('ref_axis',(-0.995256847821609,0.,0.097282099402691));
#25385=DIRECTION('center_axis',(0.,-1.,0.));
#25386=DIRECTION('ref_axis',(-0.995256847821544,0.,0.0972820994033555));
#25387=DIRECTION('',(0.,1.,0.));
#25388=DIRECTION('center_axis',(0.,1.,0.));
#25389=DIRECTION('ref_axis',(-0.995256847821544,0.,0.0972820994033555));
#25390=DIRECTION('center_axis',(0.,-1.,0.));
#25391=DIRECTION('ref_axis',(-0.589552929365356,0.,0.807729746559286));
#25392=DIRECTION('center_axis',(0.,1.,0.));
#25393=DIRECTION('ref_axis',(-0.589552929372405,0.,0.807729746554141));
#25394=DIRECTION('',(0.,-1.,0.));
#25395=DIRECTION('center_axis',(0.,-1.,0.));
#25396=DIRECTION('ref_axis',(-0.589552929372405,0.,0.807729746554141));
#25397=DIRECTION('center_axis',(0.163624134736254,0.,0.986522753174914));
#25398=DIRECTION('ref_axis',(0.,-1.,0.));
#25399=DIRECTION('',(-0.986522753174779,0.,0.163624134737066));
#25400=DIRECTION('',(0.,1.,0.));
#25401=DIRECTION('',(0.986522753174779,0.,-0.163624134737066));
#25402=DIRECTION('center_axis',(0.,-1.,0.));
#25403=DIRECTION('ref_axis',(-0.853780676609419,0.,-0.520632842076221));
#25404=DIRECTION('center_axis',(0.,1.,0.));
#25405=DIRECTION('ref_axis',(-0.853780676602481,0.,-0.520632842087598));
#25406=DIRECTION('',(0.,-1.,0.));
#25407=DIRECTION('center_axis',(0.,-1.,0.));
#25408=DIRECTION('ref_axis',(-0.853780676602481,0.,-0.520632842087598));
#25409=DIRECTION('',(0.,1.,0.));
#25410=DIRECTION('center_axis',(0.,-1.,0.));
#25411=DIRECTION('ref_axis',(-0.974044425513625,0.,0.22635692418354));
#25412=DIRECTION('center_axis',(0.,-1.,0.));
#25413=DIRECTION('ref_axis',(-0.974044425513499,0.,0.226356924184081));
#25414=DIRECTION('',(0.,1.,0.));
#25415=DIRECTION('center_axis',(0.,1.,0.));
#25416=DIRECTION('ref_axis',(-0.974044425513499,0.,0.226356924184081));
#25417=DIRECTION('center_axis',(0.,-1.,0.));
#25418=DIRECTION('ref_axis',(-0.479079334165918,0.,0.877771605587206));
#25419=DIRECTION('center_axis',(0.,1.,0.));
#25420=DIRECTION('ref_axis',(-0.479079334179917,0.,0.877771605579565));
#25421=DIRECTION('',(0.,-1.,0.));
#25422=DIRECTION('center_axis',(0.,-1.,0.));
#25423=DIRECTION('ref_axis',(-0.479079334179917,0.,0.877771605579565));
#25424=DIRECTION('center_axis',(0.290991366091359,0.,0.956725679001188));
#25425=DIRECTION('ref_axis',(0.,-1.,0.));
#25426=DIRECTION('',(-0.956725679000994,0.,0.290991366091996));
#25427=DIRECTION('',(0.,1.,0.));
#25428=DIRECTION('',(0.956725679000994,0.,-0.290991366091996));
#25429=DIRECTION('center_axis',(-0.22635692418354,0.,-0.974044425513625));
#25430=DIRECTION('ref_axis',(-0.974044425513625,0.,0.22635692418354));
#25431=DIRECTION('',(-0.974044425513455,0.,0.226356924184268));
#25432=DIRECTION('',(0.,-1.,0.));
#25433=DIRECTION('',(0.974044425513455,0.,-0.226356924184268));
#25434=DIRECTION('center_axis',(-0.0972820994026909,0.,-0.995256847821609));
#25435=DIRECTION('ref_axis',(-0.995256847821609,0.,0.0972820994026909));
#25436=DIRECTION('',(-0.995256847821521,0.,0.0972820994035846));
#25437=DIRECTION('',(0.,-1.,0.));
#25438=DIRECTION('',(0.995256847821521,0.,-0.0972820994035846));
#25439=DIRECTION('center_axis',(0.163624134736254,0.,-0.986522753174914));
#25440=DIRECTION('ref_axis',(0.,-1.,0.));
#25441=DIRECTION('',(-0.986522753174779,0.,-0.163624134737066));
#25442=DIRECTION('',(0.,-1.,0.));
#25443=DIRECTION('',(0.986522753174779,0.,0.163624134737066));
#25444=DIRECTION('center_axis',(0.290991366091358,0.,-0.956725679001189));
#25445=DIRECTION('ref_axis',(0.,-1.,0.));
#25446=DIRECTION('',(-0.956725679000995,0.,-0.290991366091995));
#25447=DIRECTION('',(0.,-1.,0.));
#25448=DIRECTION('',(0.956725679000995,0.,0.290991366091995));
#25449=DIRECTION('center_axis',(0.,1.,0.));
#25450=DIRECTION('ref_axis',(0.942641491092178,0.,0.333806859233771));
#25451=DIRECTION('center_axis',(0.,-1.,0.));
#25452=DIRECTION('ref_axis',(0.942641491092022,0.,0.333806859234212));
#25453=DIRECTION('',(0.,-1.,0.));
#25454=DIRECTION('center_axis',(0.,1.,0.));
#25455=DIRECTION('ref_axis',(0.942641491092022,0.,0.333806859234212));
#25456=DIRECTION('center_axis',(0.,1.,0.));
#25457=DIRECTION('ref_axis',(0.942641491092178,0.,0.333806859233771));
#25458=DIRECTION('center_axis',(0.,1.,0.));
#25459=DIRECTION('ref_axis',(0.942641491092022,0.,0.333806859234212));
#25460=DIRECTION('center_axis',(0.,-1.,0.));
#25461=DIRECTION('ref_axis',(0.942641491092022,0.,0.333806859234212));
#25462=DIRECTION('center_axis',(0.,1.,0.));
#25463=DIRECTION('ref_axis',(1.,0.,0.));
#25464=DIRECTION('',(-0.942641491091975,0.,0.333806859234346));
#25465=DIRECTION('center_axis',(0.,-1.,0.));
#25466=DIRECTION('ref_axis',(-0.942641491092032,0.,-0.333806859234184));
#25467=DIRECTION('',(0.942641491091975,0.,0.333806859234345));
#25468=DIRECTION('center_axis',(0.,1.,0.));
#25469=DIRECTION('ref_axis',(0.942641491092022,0.,0.333806859234212));
#25470=DIRECTION('center_axis',(0.,1.,0.));
#25471=DIRECTION('ref_axis',(0.942641491092022,0.,0.333806859234212));
#25472=DIRECTION('center_axis',(0.,1.,0.));
#25473=DIRECTION('ref_axis',(0.942641491092022,0.,0.333806859234212));
#25474=DIRECTION('',(-0.999440149526004,0.,-0.0334572490715973));
#25475=DIRECTION('center_axis',(0.,1.,0.));
#25476=DIRECTION('ref_axis',(0.942641491092022,0.,0.333806859234212));
#25477=DIRECTION('center_axis',(0.,1.,0.));
#25478=DIRECTION('ref_axis',(0.942641491092178,0.,0.333806859233771));
#25479=DIRECTION('center_axis',(0.,-1.,0.));
#25480=DIRECTION('ref_axis',(0.942641491092022,0.,0.333806859234212));
#25481=DIRECTION('',(0.,-1.,0.));
#25482=DIRECTION('center_axis',(0.,1.,0.));
#25483=DIRECTION('ref_axis',(0.942641491092178,0.,0.333806859233771));
#25484=DIRECTION('',(0.,1.,0.));
#25485=DIRECTION('center_axis',(0.,-1.,0.));
#25486=DIRECTION('ref_axis',(0.942641491092022,0.,0.333806859234212));
#25487=DIRECTION('center_axis',(0.0334572490706318,0.,-0.999440149526036));
#25488=DIRECTION('ref_axis',(0.,-1.,0.));
#25489=DIRECTION('',(0.999440149526004,0.,0.0334572490715973));
#25490=DIRECTION('center_axis',(0.,1.,0.));
#25491=DIRECTION('ref_axis',(0.942641491092178,0.,0.333806859233771));
#25492=DIRECTION('center_axis',(0.,-1.,0.));
#25493=DIRECTION('ref_axis',(0.942641491092022,0.,0.333806859234212));
#25494=DIRECTION('center_axis',(0.333806859233772,0.,0.942641491092178));
#25495=DIRECTION('ref_axis',(0.,-1.,0.));
#25496=DIRECTION('',(0.942641491091975,0.,-0.333806859234346));
#25497=DIRECTION('',(0.,1.,0.));
#25498=DIRECTION('center_axis',(0.,1.,0.));
#25499=DIRECTION('ref_axis',(-0.942641491092178,0.,-0.333806859233771));
#25500=DIRECTION('center_axis',(0.,1.,0.));
#25501=DIRECTION('ref_axis',(-0.942641491092032,0.,-0.333806859234184));
#25502=DIRECTION('',(0.,1.,0.));
#25503=DIRECTION('center_axis',(0.333806859233771,0.,-0.942641491092178));
#25504=DIRECTION('ref_axis',(0.,-1.,0.));
#25505=DIRECTION('',(-0.942641491091975,0.,-0.333806859234345));
#25506=DIRECTION('center_axis',(0.,1.,0.));
#25507=DIRECTION('ref_axis',(0.942641491092178,0.,0.333806859233771));
#25508=DIRECTION('center_axis',(0.,-1.,0.));
#25509=DIRECTION('ref_axis',(0.942641491092022,0.,0.333806859234212));
#25510=DIRECTION('center_axis',(0.,1.,0.));
#25511=DIRECTION('ref_axis',(1.,0.,0.));
#31596=CARTESIAN_POINT('',(0.,0.,0.));
#31597=CARTESIAN_POINT('Origin',(-0.0126992616256242,-0.008,-0.00360121565085291));
#31598=CARTESIAN_POINT('',(-0.0126265137841014,-0.008,-0.00384039707060321));
#31599=CARTESIAN_POINT('',(-0.0129397779442914,-0.008,-0.00366942049272513));
#31600=CARTESIAN_POINT('Origin',(-0.0126992616256342,-0.00799999999999,
-0.00360121565086291));
#31601=CARTESIAN_POINT('',(-0.0129397779442914,-0.024,-0.00366942049272513));
#31602=CARTESIAN_POINT('',(-0.0129397779443014,-0.00799999999999,-0.00366942049273513));
#31603=CARTESIAN_POINT('',(-0.0126265137841014,-0.024,-0.00384039707060321));
#31604=CARTESIAN_POINT('Origin',(-0.0126992616256342,-0.02400000000001,
-0.00360121565086291));
#31605=CARTESIAN_POINT('',(-0.0126265137841114,-0.00799999999999,-0.00384039707061321));
#31606=CARTESIAN_POINT('Origin',(-4.44089209850063E-17,-0.008,6.72997231505748E-33));
#31607=CARTESIAN_POINT('',(-0.0130408866654485,-0.008,-0.0032920776082785));
#31608=CARTESIAN_POINT('Origin',(-4.44089209850063E-17,-0.00799999999999,
6.72997231505748E-33));
#31609=CARTESIAN_POINT('',(-0.0130408866654485,-0.024,-0.0032920776082785));
#31610=CARTESIAN_POINT('',(-0.0130408866654585,-0.00799999999999,-0.0032920776082885));
#31611=CARTESIAN_POINT('Origin',(-4.44089209850063E-17,-0.02400000000001,
6.72997231505748E-33));
#31612=CARTESIAN_POINT('Origin',(-0.0127984910025219,-0.008,-0.00323088657466738));
#31613=CARTESIAN_POINT('',(-0.0128550802335678,-0.008,-0.00298737546828897));
#31614=CARTESIAN_POINT('Origin',(-0.0127984910025319,-0.00799999999999,
-0.00323088657467738));
#31615=CARTESIAN_POINT('',(-0.0128550802335678,-0.024,-0.00298737546828897));
#31616=CARTESIAN_POINT('',(-0.0128550802335778,-0.00799999999999,-0.00298737546829897));
#31617=CARTESIAN_POINT('Origin',(-0.0127984910025319,-0.02400000000001,
-0.00323088657467738));
#31618=CARTESIAN_POINT('Origin',(-0.0126625775316771,-0.008,-0.00294264001438602));
#31619=CARTESIAN_POINT('',(-0.0126625775316771,-0.008,-0.00294264001438602));
#31620=CARTESIAN_POINT('',(-0.0125348531511851,-0.00799999999999,-0.00291295831081412));
#31621=CARTESIAN_POINT('',(-0.0126625775316771,-0.024,-0.00294264001438602));
#31622=CARTESIAN_POINT('',(-0.0126625775316871,-0.016,-0.00294264001439602));
#31623=CARTESIAN_POINT('',(-0.0125348531511851,-0.02400000000001,-0.00291295831081412));
#31624=CARTESIAN_POINT('Origin',(-0.0130606706482359,-0.008,-0.00191282048773811));
#31625=CARTESIAN_POINT('',(-0.0130197646145518,-0.008,-0.00215945117603184));
#31626=CARTESIAN_POINT('',(-0.0133080318347555,-0.008,-0.00194904814849073));
#31627=CARTESIAN_POINT('Origin',(-0.0130606706482459,-0.00799999999999,
-0.00191282048774811));
#31628=CARTESIAN_POINT('',(-0.0133080318347555,-0.024,-0.00194904814849073));
#31629=CARTESIAN_POINT('',(-0.0133080318347655,-0.00799999999999,-0.00194904814850073));
#31630=CARTESIAN_POINT('',(-0.0130197646145518,-0.024,-0.00215945117603184));
#31631=CARTESIAN_POINT('Origin',(-0.0130606706482459,-0.02400000000001,
-0.00191282048774811));
#31632=CARTESIAN_POINT('',(-0.0130197646145618,-0.00799999999999,-0.00215945117604184));
#31633=CARTESIAN_POINT('Origin',(-4.44089209850063E-17,-0.008,6.72997231505748E-33));
#31634=CARTESIAN_POINT('',(-0.0133590224269186,-0.008,-0.00156173614835727));
#31635=CARTESIAN_POINT('Origin',(-4.44089209850063E-17,-0.00799999999999,
6.72997231505748E-33));
#31636=CARTESIAN_POINT('',(-0.0133590224269186,-0.024,-0.00156173614835727));
#31637=CARTESIAN_POINT('',(-0.0133590224269286,-0.00799999999999,-0.00156173614836727));
#31638=CARTESIAN_POINT('Origin',(-4.44089209850063E-17,-0.02400000000001,
6.72997231505748E-33));
#31639=CARTESIAN_POINT('Origin',(-0.0131107134598755,-0.008,-0.00153270759541383));
#31640=CARTESIAN_POINT('',(-0.0131350339847262,-0.008,-0.00128389338345842));
#31641=CARTESIAN_POINT('Origin',(-0.0131107134598855,-0.00799999999999,
-0.00153270759542383));
#31642=CARTESIAN_POINT('',(-0.0131350339847262,-0.024,-0.00128389338345842));
#31643=CARTESIAN_POINT('',(-0.0131350339847362,-0.00799999999999,-0.00128389338346842));
#31644=CARTESIAN_POINT('Origin',(-0.0131107134598855,-0.02400000000001,
-0.00153270759542383));
#31645=CARTESIAN_POINT('Origin',(-0.0129383390216809,-0.008,-0.00126466729223498));
#31646=CARTESIAN_POINT('',(-0.0129383390216809,-0.008,-0.00126466729223498));
#31647=CARTESIAN_POINT('',(-0.0129458744527519,-0.00799999999999,-0.00126540384839641));
#31648=CARTESIAN_POINT('',(-0.0129383390216809,-0.024,-0.00126466729223498));
#31649=CARTESIAN_POINT('',(-0.0129383390216909,-0.016,-0.00126466729224498));
#31650=CARTESIAN_POINT('',(-0.0129458744527519,-0.02400000000001,-0.00126540384839641));
#31651=CARTESIAN_POINT('Origin',(-0.0131986079749541,-0.008,-0.000191696435744077));
#31652=CARTESIAN_POINT('',(-0.0131902436626865,-0.008,-0.000441556473125586));
#31653=CARTESIAN_POINT('',(-0.0134485816108434,-0.008,-0.000195327050057411));
#31654=CARTESIAN_POINT('Origin',(-0.0131986079749641,-0.00799999999999,
-0.000191696435754077));
#31655=CARTESIAN_POINT('',(-0.0134485816108434,-0.024,-0.000195327050057411));
#31656=CARTESIAN_POINT('',(-0.0134485816108534,-0.00799999999999,-0.000195327050067411));
#31657=CARTESIAN_POINT('',(-0.0131902436626865,-0.024,-0.000441556473125586));
#31658=CARTESIAN_POINT('Origin',(-0.0131986079749641,-0.02400000000001,
-0.000191696435754077));
#31659=CARTESIAN_POINT('',(-0.0131902436626965,-0.00799999999999,-0.000441556473135586));
#31660=CARTESIAN_POINT('Origin',(-4.44089209850063E-17,-0.008,6.72997231505748E-33));
#31661=CARTESIAN_POINT('',(-0.0134485816108434,-0.008,0.000195327050057416));
#31662=CARTESIAN_POINT('Origin',(-4.44089209850063E-17,-0.00799999999999,
6.72997231505748E-33));
#31663=CARTESIAN_POINT('',(-0.0134485816108434,-0.024,0.000195327050057416));
#31664=CARTESIAN_POINT('',(-0.0134485816108534,-0.00799999999999,0.000195327050067416));
#31665=CARTESIAN_POINT('Origin',(-4.44089209850063E-17,-0.02400000000001,
6.72997231505748E-33));
#31666=CARTESIAN_POINT('Origin',(-0.0131986079749541,-0.008,0.000191696435744081));
#31667=CARTESIAN_POINT('',(-0.0131902436626865,-0.008,0.00044155647312559));
#31668=CARTESIAN_POINT('Origin',(-0.0131986079749641,-0.00799999999999,
0.000191696435754081));
#31669=CARTESIAN_POINT('',(-0.0131902436626865,-0.024,0.00044155647312559));
#31670=CARTESIAN_POINT('',(-0.0131902436626965,-0.00799999999999,0.00044155647313559));
#31671=CARTESIAN_POINT('Origin',(-0.0131986079749641,-0.02400000000001,
0.000191696435754081));
#31672=CARTESIAN_POINT('Origin',(-0.0129927219438385,-0.008,0.000434944237918218));
#31673=CARTESIAN_POINT('',(-0.0129927219438385,-0.008,0.000434944237918218));
#31674=CARTESIAN_POINT('',(-0.0130276266077339,-0.00799999999999,0.000436112706129036));
#31675=CARTESIAN_POINT('',(-0.0129927219438385,-0.024,0.000434944237918218));
#31676=CARTESIAN_POINT('',(-0.0129927219438485,-0.016,0.000434944237928218));
#31677=CARTESIAN_POINT('',(-0.0130276266077339,-0.02400000000001,0.000436112706129036));
#31678=CARTESIAN_POINT('Origin',(-0.0131107134598755,-0.008,0.00153270759541383));
#31679=CARTESIAN_POINT('',(-0.0131350339847262,-0.008,0.00128389338345843));
#31680=CARTESIAN_POINT('',(-0.0133590224269186,-0.008,0.00156173614835727));
#31681=CARTESIAN_POINT('Origin',(-0.0131107134598855,-0.00799999999999,
0.00153270759542383));
#31682=CARTESIAN_POINT('',(-0.0133590224269186,-0.024,0.00156173614835727));
#31683=CARTESIAN_POINT('',(-0.0133590224269286,-0.00799999999999,0.00156173614836727));
#31684=CARTESIAN_POINT('',(-0.0131350339847262,-0.024,0.00128389338345843));
#31685=CARTESIAN_POINT('Origin',(-0.0131107134598855,-0.02400000000001,
0.00153270759542383));
#31686=CARTESIAN_POINT('',(-0.0131350339847362,-0.00799999999999,0.00128389338346843));
#31687=CARTESIAN_POINT('Origin',(-4.44089209850063E-17,-0.008,6.72997231505748E-33));
#31688=CARTESIAN_POINT('',(-0.0133080318347555,-0.008,0.00194904814849073));
#31689=CARTESIAN_POINT('Origin',(-4.44089209850063E-17,-0.00799999999999,
6.72997231505748E-33));
#31690=CARTESIAN_POINT('',(-0.0133080318347555,-0.024,0.00194904814849073));
#31691=CARTESIAN_POINT('',(-0.0133080318347655,-0.00799999999999,0.00194904814850073));
#31692=CARTESIAN_POINT('Origin',(-4.44089209850063E-17,-0.02400000000001,
6.72997231505748E-33));
#31693=CARTESIAN_POINT('Origin',(-0.0130606706482359,-0.008,0.00191282048773811));
#31694=CARTESIAN_POINT('',(-0.0130197646145518,-0.008,0.00215945117603184));
#31695=CARTESIAN_POINT('Origin',(-0.0130606706482459,-0.00799999999999,
0.00191282048774811));
#31696=CARTESIAN_POINT('',(-0.0130197646145518,-0.024,0.00215945117603184));
#31697=CARTESIAN_POINT('',(-0.0130197646145618,-0.00799999999999,0.00215945117604184));
#31698=CARTESIAN_POINT('Origin',(-0.0130606706482459,-0.02400000000001,
0.00191282048774811));
#31699=CARTESIAN_POINT('Origin',(-0.0128247957912739,-0.008,0.00212711375157131));
#31700=CARTESIAN_POINT('',(-0.0128247957912739,-0.008,0.00212711375157131));
#31701=CARTESIAN_POINT('',(-0.0127759261415696,-0.00799999999999,0.00211900825769013));
#31702=CARTESIAN_POINT('',(-0.0128247957912739,-0.024,0.00212711375157131));
#31703=CARTESIAN_POINT('',(-0.0128247957912839,-0.016,0.00212711375158131));
#31704=CARTESIAN_POINT('',(-0.0127759261415696,-0.02400000000001,0.00211900825769013));
#31705=CARTESIAN_POINT('Origin',(-0.0127984910025219,-0.008,0.00323088657466738));
#31706=CARTESIAN_POINT('',(-0.0128550802335678,-0.008,0.00298737546828897));
#31707=CARTESIAN_POINT('',(-0.0130408866654485,-0.008,0.0032920776082785));
#31708=CARTESIAN_POINT('Origin',(-0.0127984910025319,-0.00799999999999,
0.00323088657467738));
#31709=CARTESIAN_POINT('',(-0.0130408866654485,-0.024,0.0032920776082785));
#31710=CARTESIAN_POINT('',(-0.0130408866654585,-0.00799999999999,0.0032920776082885));
#31711=CARTESIAN_POINT('',(-0.0128550802335678,-0.024,0.00298737546828897));
#31712=CARTESIAN_POINT('Origin',(-0.0127984910025319,-0.02400000000001,
0.00323088657467738));
#31713=CARTESIAN_POINT('',(-0.0128550802335778,-0.00799999999999,0.00298737546829897));
#31714=CARTESIAN_POINT('Origin',(-4.44089209850063E-17,-0.008,6.72997231505748E-33));
#31715=CARTESIAN_POINT('',(-0.0129397779442914,-0.008,0.00366942049272513));
#31716=CARTESIAN_POINT('Origin',(-4.44089209850063E-17,-0.00799999999999,
6.72997231505748E-33));
#31717=CARTESIAN_POINT('',(-0.0129397779442914,-0.024,0.00366942049272513));
#31718=CARTESIAN_POINT('',(-0.0129397779443014,-0.00799999999999,0.00366942049273513));
#31719=CARTESIAN_POINT('Origin',(-4.44089209850063E-17,-0.02400000000001,
6.72997231505748E-33));
#31720=CARTESIAN_POINT('Origin',(-0.0126992616256242,-0.008,0.00360121565085292));
#31721=CARTESIAN_POINT('',(-0.0126265137841014,-0.008,0.00384039707060321));
#31722=CARTESIAN_POINT('Origin',(-0.0126992616256342,-0.00799999999999,
0.00360121565086292));
#31723=CARTESIAN_POINT('',(-0.0126265137841014,-0.024,0.00384039707060321));
#31724=CARTESIAN_POINT('',(-0.0126265137841114,-0.00799999999999,0.00384039707061321));
#31725=CARTESIAN_POINT('Origin',(-0.0126992616256342,-0.02400000000001,
0.00360121565086292));
#31726=CARTESIAN_POINT('Origin',(-0.0124374338270155,-0.008,0.00378288775918766));
#31727=CARTESIAN_POINT('',(-0.0124374338270155,-0.008,0.00378288775918766));
#31728=CARTESIAN_POINT('',(-0.0122036407116943,-0.00799999999999,0.00371177878877263));
#31729=CARTESIAN_POINT('',(-0.0124374338270155,-0.024,0.00378288775918766));
#31730=CARTESIAN_POINT('',(-0.0124374338270255,-0.016,0.00378288775919766));
#31731=CARTESIAN_POINT('',(-0.0122036407116943,-0.02400000000001,0.00371177878877263));
#31732=CARTESIAN_POINT('Origin',(-0.0131008975231583,-0.008,0.00304450063026861));
#31733=CARTESIAN_POINT('',(-0.0126625775316771,-0.024,0.00294264001438602));
#31734=CARTESIAN_POINT('',(-0.0127540131469256,-0.02400000000001,0.00296388861875542));
#31735=CARTESIAN_POINT('',(-0.0126625775316771,-0.008,0.00294264001438602));
#31736=CARTESIAN_POINT('',(-0.0126625775316871,-0.016,0.00294264001439602));
#31737=CARTESIAN_POINT('',(-0.0127540131469256,-0.00799999999999,0.00296388861875542));
#31738=CARTESIAN_POINT('Origin',(-0.0133862046032006,-0.008,0.00130844423696619));
#31739=CARTESIAN_POINT('',(-0.0129383390216809,-0.024,0.00126466729223498));
#31740=CARTESIAN_POINT('',(-0.0131698072435117,-0.02400000000001,0.00128729232076202));
#31741=CARTESIAN_POINT('',(-0.0129383390216809,-0.008,0.00126466729223498));
#31742=CARTESIAN_POINT('',(-0.0129383390216909,-0.016,0.00126466729224498));
#31743=CARTESIAN_POINT('',(-0.0131698072435117,-0.00799999999999,0.00128729232076202));
#31744=CARTESIAN_POINT('Origin',(-0.0132687310302026,-0.008,-0.00220074461220262));
#31745=CARTESIAN_POINT('',(-0.0128247957912739,-0.024,-0.0021271137515713));
#31746=CARTESIAN_POINT('',(-0.0129978937610339,-0.02400000000001,-0.00215582368800578));
#31747=CARTESIAN_POINT('',(-0.0128247957912739,-0.008,-0.0021271137515713));
#31748=CARTESIAN_POINT('',(-0.0128247957912839,-0.016,-0.0021271137515813));
#31749=CARTESIAN_POINT('',(-0.0129978937610339,-0.00799999999999,-0.00215582368800578));
#31750=CARTESIAN_POINT('Origin',(-0.012867960382566,-0.008,-0.00391383387392877));
#31751=CARTESIAN_POINT('',(-0.0124374338270155,-0.024,-0.00378288775918766));
#31752=CARTESIAN_POINT('',(-0.0124189039894696,-0.02400000000001,-0.00377725184614318));
#31753=CARTESIAN_POINT('',(-0.0124374338270155,-0.008,-0.00378288775918766));
#31754=CARTESIAN_POINT('',(-0.0124374338270255,-0.016,-0.00378288775919766));
#31755=CARTESIAN_POINT('',(-0.0124189039894696,-0.00799999999999,-0.00377725184614318));
#31756=CARTESIAN_POINT('Origin',(-4.44089209850063E-17,-0.016,6.72997231505748E-33));
#31757=CARTESIAN_POINT('',(-0.0122543393841983,-0.008,0.00433948917003902));
#31758=CARTESIAN_POINT('Origin',(-4.44089209850063E-17,-0.00799999999999,
6.72997231505748E-33));
#31759=CARTESIAN_POINT('',(-0.0122543393841983,-0.024,0.00433948917003902));
#31760=CARTESIAN_POINT('',(-0.0122543393842083,-0.016,0.00433948917004902));
#31761=CARTESIAN_POINT('Origin',(-4.44089209850063E-17,-0.02400000000001,
6.72997231505748E-33));
#31762=CARTESIAN_POINT('Origin',(-4.44089209850063E-17,-0.016,6.72997231505748E-33));
#31763=CARTESIAN_POINT('Origin',(-4.44089209850063E-17,-0.02400000000001,
6.72997231505748E-33));
#31764=CARTESIAN_POINT('Origin',(-4.44089209850063E-17,-0.00799999999999,
6.72997231505748E-33));
#31765=CARTESIAN_POINT('Origin',(-0.0130771696920992,-0.024,1.11022302462517E-18));
#31766=CARTESIAN_POINT('',(-0.0131027167261813,-0.024,0.00463991534334942));
#31767=CARTESIAN_POINT('',(-0.0131027167261913,-0.02400000000001,0.00463991534335942));
#31768=CARTESIAN_POINT('',(-0.0131027167261813,-0.024,-0.00463991534334942));
#31769=CARTESIAN_POINT('Origin',(-4.44089209850063E-17,-0.02400000000001,
6.72997231505748E-33));
#31770=CARTESIAN_POINT('',(-0.0122543393841983,-0.024,-0.00433948917003902));
#31771=CARTESIAN_POINT('',(-0.0122543393842083,-0.02400000000001,-0.00433948917004902));
#31772=CARTESIAN_POINT('Origin',(-4.44089209850063E-17,-0.02400000000001,
6.72997231505748E-33));
#31773=CARTESIAN_POINT('Origin',(-4.44089209850063E-17,-0.02400000000001,
6.72997231505748E-33));
#31774=CARTESIAN_POINT('',(-0.0129927219438385,-0.024,-0.000434944237918213));
#31775=CARTESIAN_POINT('Origin',(-4.44089209850063E-17,-0.02400000000001,
6.72997231505748E-33));
#31776=CARTESIAN_POINT('',(-0.0132525006413773,-0.02400000000001,-0.000443640587169925));
#31777=CARTESIAN_POINT('Origin',(-4.44089209850063E-17,-0.02400000000001,
6.72997231505748E-33));
#31778=CARTESIAN_POINT('Origin',(-4.44089209850063E-17,-0.016,6.72997231505748E-33));
#31779=CARTESIAN_POINT('',(-0.0129927219438385,-0.008,-0.000434944237918213));
#31780=CARTESIAN_POINT('Origin',(-4.44089209850063E-17,-0.00799999999999,
6.72997231505748E-33));
#31781=CARTESIAN_POINT('',(-0.0129927219438485,-0.016,-0.000434944237928214));
#31782=CARTESIAN_POINT('Origin',(-4.44089209850063E-17,-0.016,6.72997231505748E-33));
#31783=CARTESIAN_POINT('',(-0.0122543393841983,-0.008,-0.00433948917003902));
#31784=CARTESIAN_POINT('',(-0.0122543393842083,-0.016,-0.00433948917004902));
#31785=CARTESIAN_POINT('Origin',(-4.44089209850063E-17,-0.00799999999999,
6.72997231505748E-33));
#31786=CARTESIAN_POINT('Origin',(-0.0134424700111252,-0.008,-0.00045));
#31787=CARTESIAN_POINT('',(-0.0132525006413773,-0.00799999999999,-0.000443640587169925));
#31788=CARTESIAN_POINT('Origin',(-4.44089209850063E-17,-0.016,6.72997231505748E-33));
#31789=CARTESIAN_POINT('Origin',(-4.44089209850063E-17,-0.00799999999999,
6.72997231505748E-33));
#31790=CARTESIAN_POINT('Origin',(-0.0131027167261813,-0.016,0.00463991534334942));
#31791=CARTESIAN_POINT('',(-0.0131027167261813,-0.008,0.00463991534334942));
#31792=CARTESIAN_POINT('',(-0.0131027167261913,-0.00799999999999,0.00463991534335942));
#31793=CARTESIAN_POINT('',(-0.0131027167261913,-0.016,0.00463991534335942));
#31794=CARTESIAN_POINT('Origin',(-4.44089209850063E-17,-0.016,6.72997231505748E-33));
#31795=CARTESIAN_POINT('',(-0.0131027167261813,-0.008,-0.00463991534334942));
#31796=CARTESIAN_POINT('Origin',(-4.44089209850063E-17,-0.00799999999999,
6.72997231505748E-33));
#31797=CARTESIAN_POINT('',(-0.0131027167261913,-0.016,-0.00463991534335942));
#31798=CARTESIAN_POINT('Origin',(-0.0122543393841983,-0.016,-0.00433948917003902));
#31799=CARTESIAN_POINT('',(-0.0122543393842083,-0.00799999999999,-0.00433948917004902));
#31800=CARTESIAN_POINT('Origin',(-4.44089209850063E-17,-0.016,6.72997231505748E-33));
#31801=CARTESIAN_POINT('Origin',(-4.44089209850063E-17,-0.00799999999999,
6.72997231505748E-33));
#31802=CARTESIAN_POINT('Origin',(-0.0130771696920992,-0.008,1.11022302462517E-18));
#34820=UNCERTAINTY_MEASURE_WITH_UNIT(LENGTH_MEASURE(1.E-5),#34877,
'DISTANCE_ACCURACY_VALUE',
'Maximum model space distance between geometric entities at asserted c
onnectivities');
#34841=UNCERTAINTY_MEASURE_WITH_UNIT(LENGTH_MEASURE(1.E-5),#34877,
'DISTANCE_ACCURACY_VALUE',
'Maximum model space distance between geometric entities at asserted c
onnectivities');
#34855=(
GEOMETRIC_REPRESENTATION_CONTEXT(3)
GLOBAL_UNCERTAINTY_ASSIGNED_CONTEXT((#34820))
GLOBAL_UNIT_ASSIGNED_CONTEXT((#34877,#34878,#34879))
REPRESENTATION_CONTEXT('','3D')
);
#34876=(
GEOMETRIC_REPRESENTATION_CONTEXT(3)
GLOBAL_UNCERTAINTY_ASSIGNED_CONTEXT((#34841))
GLOBAL_UNIT_ASSIGNED_CONTEXT((#34877,#34878,#34879))
REPRESENTATION_CONTEXT('','3D')
);
#34877=(
LENGTH_UNIT()
NAMED_UNIT(*)
SI_UNIT($,.METRE.)
);
#34878=(
NAMED_UNIT(*)
PLANE_ANGLE_UNIT()
SI_UNIT($,.RADIAN.)
);
#34879=(
NAMED_UNIT(*)
SI_UNIT($,.STERADIAN.)
SOLID_ANGLE_UNIT()
);
#34893=SHAPE_DEFINITION_REPRESENTATION(#34927,#34997);
#34927=PRODUCT_DEFINITION_SHAPE('',$,#35032);
#34997=SHAPE_REPRESENTATION('',(#21089),#34855);
#35018=PRODUCT_DEFINITION_CONTEXT('part definition',#35122,'design');
#35032=PRODUCT_DEFINITION('Motor Stator Face 3','Motor Stator Face 3',#35066,
#35018);
#35066=PRODUCT_DEFINITION_FORMATION('',$,#35137);
#35122=APPLICATION_CONTEXT('Managed model based 3d engineering');
#35123=PRODUCT_CONTEXT('part definition',#35122,'mechanical');
#35137=PRODUCT('Motor Stator Face 3','Motor Stator Face 3',
'LEGAL AND USAGE DISCLAIMER: this Data/Model is provided \X2\201C\X0\A
S IS\X2\201D\X0\ for informational and representational only. It is a 
geometric approximation and is NOT engineered, certified, or guarantee
d for dimensional accuracy, exact tolerances, or production-level prec
ision. Vendor disclaims all implied warranties including fitness for a
 particular purpose. DO NOT USE FOR DIRECT PHYSICAL MANUFACTURING, AUT
OMATED PRODUCTION, OR SAFETY-CRITICAL SYSTEMS without independent engi
neering verification and resolution of any design discrepancies.',(#35123));
#35163=PRESENTATION_STYLE_ASSIGNMENT((#35172));
#35172=SURFACE_STYLE_USAGE(.BOTH.,#35181);
#35181=SURFACE_SIDE_STYLE('',(#35190));
#35190=SURFACE_STYLE_FILL_AREA(#35199);
#35199=FILL_AREA_STYLE('Plastic - Matte (Black)',(#35208));
#35208=FILL_AREA_STYLE_COLOUR('Plastic - Matte (Black)',#35217);
#35217=COLOUR_RGB('Plastic - Matte (Black)',0.0980392156862745,0.0980392156862745,
0.0980392156862745);
ENDSEC;
END-ISO-10303-21;
